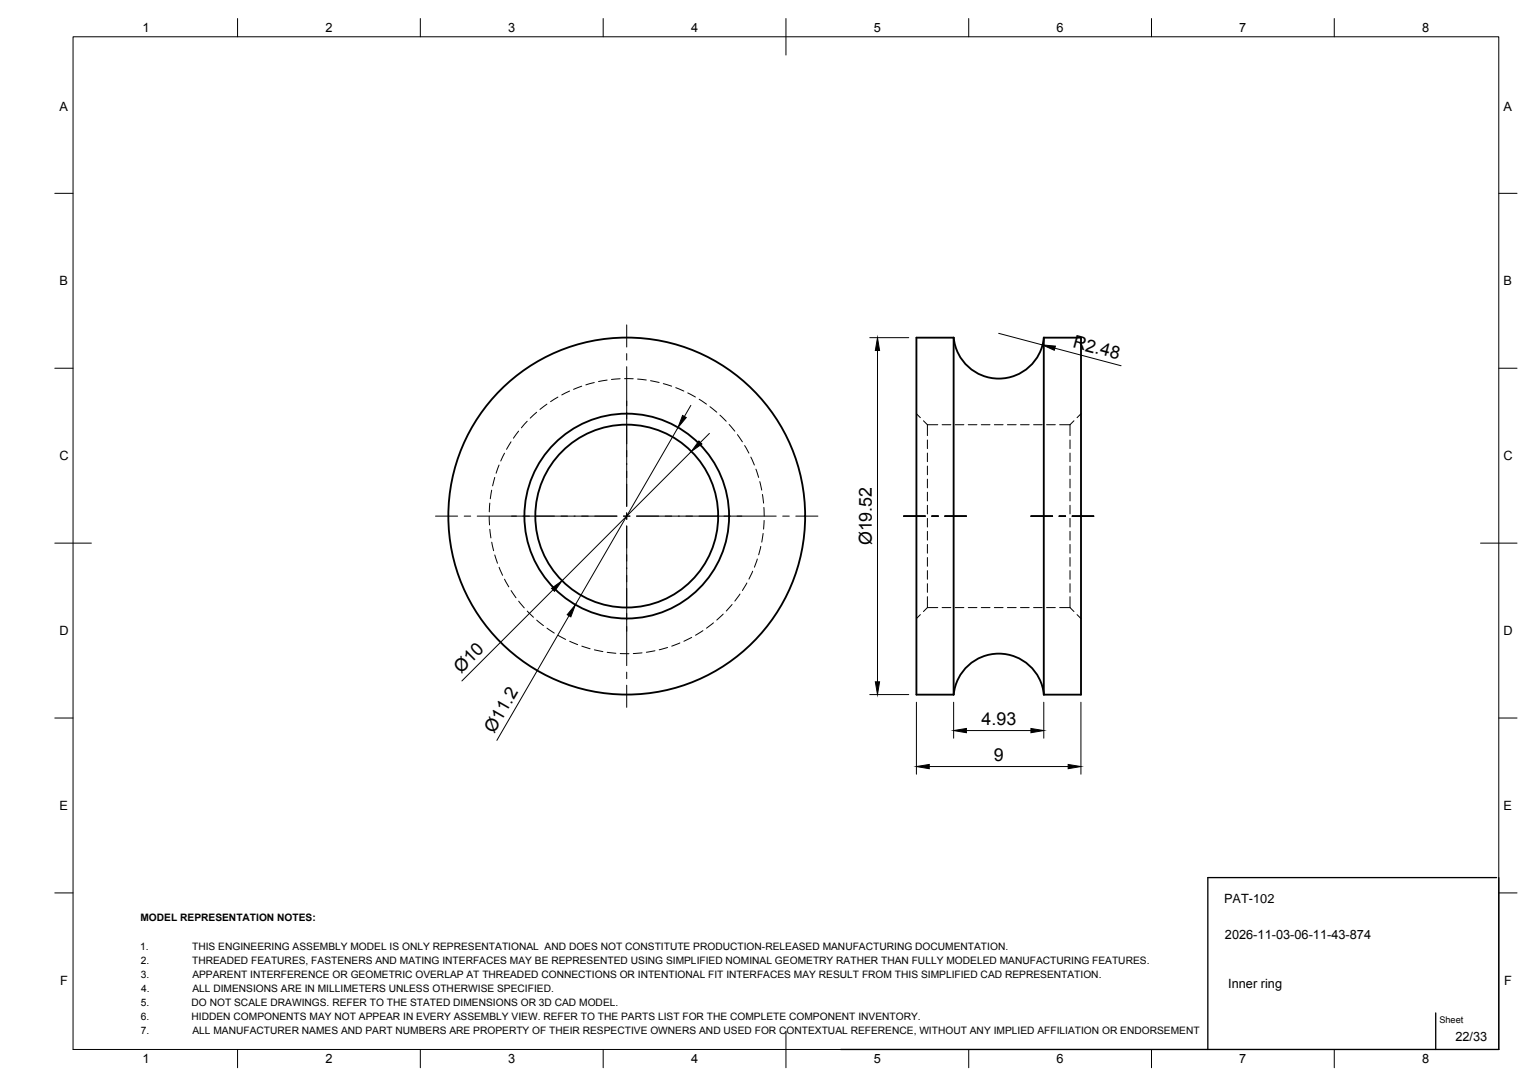
ISO-10303-21;
HEADER;
/* Generated by software containing ST-Developer
 * from STEP Tools, Inc. (www.steptools.com) 
 */

FILE_DESCRIPTION(
/* description */ ('Swing-away clamp arm'),
/* implementation_level */ '2;1');

FILE_NAME(
/* name */ 'Inner ring.step',
/* time_stamp */ '2026-10-28T03:26:03-07:00',
/* author */ (''),
/* organization */ (''),
/* preprocessor_version */ 'ST-DEVELOPER v20.2',
/* originating_system */ 'Autodesk Translation Framework v15.17.0.0',
/* authorisation */ '');

FILE_SCHEMA (('AUTOMOTIVE_DESIGN { 1 0 10303 214 3 1 1 }'));
ENDSEC;

DATA;
#10=MECHANICAL_DESIGN_GEOMETRIC_PRESENTATION_REPRESENTATION('',(#307),#10627);
#27=TOROIDAL_SURFACE('',#5581,1.,0.247676);
#204=CONICAL_SURFACE('',#5592,0.53,0.785398163397448);
#205=CONICAL_SURFACE('',#5599,0.53,0.785398163397448);
#255=SHAPE_REPRESENTATION_RELATIONSHIP('SRR','None',#10755,#281);
#281=ADVANCED_BREP_SHAPE_REPRESENTATION('',(#340),#10614);
#307=STYLED_ITEM('',(#10965),#340);
#340=MANIFOLD_SOLID_BREP('Body1',#4914);
#432=FACE_BOUND('',#1209,.T.);
#433=FACE_BOUND('',#1212,.T.);
#578=PLANE('',#5594);
#579=PLANE('',#5597);
#823=FACE_OUTER_BOUND('',#1204,.T.);
#824=FACE_OUTER_BOUND('',#1205,.T.);
#825=FACE_OUTER_BOUND('',#1206,.T.);
#826=FACE_OUTER_BOUND('',#1207,.T.);
#827=FACE_OUTER_BOUND('',#1208,.T.);
#828=FACE_OUTER_BOUND('',#1210,.T.);
#829=FACE_OUTER_BOUND('',#1211,.T.);
#830=FACE_OUTER_BOUND('',#1213,.T.);
#1204=EDGE_LOOP('',(#4041,#4042,#4043,#4044,#4045,#4046));
#1205=EDGE_LOOP('',(#4047,#4048,#4049,#4050,#4051));
#1206=EDGE_LOOP('',(#4052,#4053,#4054,#4055));
#1207=EDGE_LOOP('',(#4056,#4057,#4058,#4059));
#1208=EDGE_LOOP('',(#4060));
#1209=EDGE_LOOP('',(#4061));
#1210=EDGE_LOOP('',(#4062,#4063,#4064,#4065,#4066));
#1211=EDGE_LOOP('',(#4067));
#1212=EDGE_LOOP('',(#4068));
#1213=EDGE_LOOP('',(#4069,#4070,#4071,#4072));
#1586=LINE('',#9685,#1908);
#1587=LINE('',#9691,#1909);
#1588=LINE('',#9695,#1910);
#1589=LINE('',#9701,#1911);
#1590=LINE('',#9706,#1912);
#1908=VECTOR('',#6835,0.976185);
#1909=VECTOR('',#6842,0.5);
#1910=VECTOR('',#6847,0.53);
#1911=VECTOR('',#6856,0.976185);
#1912=VECTOR('',#6863,0.53);
#2139=CIRCLE('',#5582,0.976185);
#2140=CIRCLE('',#5583,0.976185);
#2141=CIRCLE('',#5584,0.247676);
#2142=CIRCLE('',#5585,0.976185);
#2143=CIRCLE('',#5586,0.976185);
#2144=CIRCLE('',#5588,0.976185);
#2145=CIRCLE('',#5590,0.5);
#2146=CIRCLE('',#5591,0.5);
#2147=CIRCLE('',#5593,0.56);
#2148=CIRCLE('',#5596,0.976185);
#2149=CIRCLE('',#5598,0.56);
#2514=VERTEX_POINT('',#9674);
#2515=VERTEX_POINT('',#9675);
#2516=VERTEX_POINT('',#9678);
#2517=VERTEX_POINT('',#9680);
#2518=VERTEX_POINT('',#9684);
#2519=VERTEX_POINT('',#9688);
#2520=VERTEX_POINT('',#9690);
#2521=VERTEX_POINT('',#9694);
#2522=VERTEX_POINT('',#9699);
#2523=VERTEX_POINT('',#9703);
#3053=EDGE_CURVE('',#2514,#2515,#2139,.T.);
#3054=EDGE_CURVE('',#2515,#2514,#2140,.T.);
#3055=EDGE_CURVE('',#2515,#2516,#2141,.T.);
#3056=EDGE_CURVE('',#2517,#2516,#2142,.T.);
#3057=EDGE_CURVE('',#2516,#2517,#2143,.T.);
#3058=EDGE_CURVE('',#2517,#2518,#1586,.T.);
#3059=EDGE_CURVE('',#2518,#2518,#2144,.T.);
#3060=EDGE_CURVE('',#2519,#2519,#2145,.T.);
#3061=EDGE_CURVE('',#2519,#2520,#1587,.T.);
#3062=EDGE_CURVE('',#2520,#2520,#2146,.T.);
#3063=EDGE_CURVE('',#2520,#2521,#1588,.T.);
#3064=EDGE_CURVE('',#2521,#2521,#2147,.T.);
#3065=EDGE_CURVE('',#2522,#2522,#2148,.T.);
#3066=EDGE_CURVE('',#2522,#2514,#1589,.T.);
#3067=EDGE_CURVE('',#2523,#2523,#2149,.T.);
#3068=EDGE_CURVE('',#2523,#2519,#1590,.T.);
#4041=ORIENTED_EDGE('',*,*,#3053,.F.);
#4042=ORIENTED_EDGE('',*,*,#3054,.F.);
#4043=ORIENTED_EDGE('',*,*,#3055,.T.);
#4044=ORIENTED_EDGE('',*,*,#3056,.F.);
#4045=ORIENTED_EDGE('',*,*,#3057,.F.);
#4046=ORIENTED_EDGE('',*,*,#3055,.F.);
#4047=ORIENTED_EDGE('',*,*,#3056,.T.);
#4048=ORIENTED_EDGE('',*,*,#3057,.T.);
#4049=ORIENTED_EDGE('',*,*,#3058,.T.);
#4050=ORIENTED_EDGE('',*,*,#3059,.T.);
#4051=ORIENTED_EDGE('',*,*,#3058,.F.);
#4052=ORIENTED_EDGE('',*,*,#3060,.T.);
#4053=ORIENTED_EDGE('',*,*,#3061,.T.);
#4054=ORIENTED_EDGE('',*,*,#3062,.F.);
#4055=ORIENTED_EDGE('',*,*,#3061,.F.);
#4056=ORIENTED_EDGE('',*,*,#3062,.T.);
#4057=ORIENTED_EDGE('',*,*,#3063,.T.);
#4058=ORIENTED_EDGE('',*,*,#3064,.F.);
#4059=ORIENTED_EDGE('',*,*,#3063,.F.);
#4060=ORIENTED_EDGE('',*,*,#3059,.F.);
#4061=ORIENTED_EDGE('',*,*,#3064,.T.);
#4062=ORIENTED_EDGE('',*,*,#3065,.F.);
#4063=ORIENTED_EDGE('',*,*,#3066,.T.);
#4064=ORIENTED_EDGE('',*,*,#3053,.T.);
#4065=ORIENTED_EDGE('',*,*,#3054,.T.);
#4066=ORIENTED_EDGE('',*,*,#3066,.F.);
#4067=ORIENTED_EDGE('',*,*,#3065,.T.);
#4068=ORIENTED_EDGE('',*,*,#3067,.F.);
#4069=ORIENTED_EDGE('',*,*,#3067,.T.);
#4070=ORIENTED_EDGE('',*,*,#3068,.T.);
#4071=ORIENTED_EDGE('',*,*,#3060,.F.);
#4072=ORIENTED_EDGE('',*,*,#3068,.F.);
#4559=CYLINDRICAL_SURFACE('',#5587,0.976185);
#4560=CYLINDRICAL_SURFACE('',#5589,0.5);
#4561=CYLINDRICAL_SURFACE('',#5595,0.976185);
#4778=ADVANCED_FACE('',(#823),#27,.F.);
#4779=ADVANCED_FACE('',(#824),#4559,.T.);
#4780=ADVANCED_FACE('',(#825),#4560,.F.);
#4781=ADVANCED_FACE('',(#826),#204,.F.);
#4782=ADVANCED_FACE('',(#827,#432),#578,.T.);
#4783=ADVANCED_FACE('',(#828),#4561,.T.);
#4784=ADVANCED_FACE('',(#829,#433),#579,.T.);
#4785=ADVANCED_FACE('',(#830),#205,.F.);
#4914=CLOSED_SHELL('',(#4778,#4779,#4780,#4781,#4782,#4783,#4784,#4785));
#5580=AXIS2_PLACEMENT_3D('',#9672,#6819,#6820);
#5581=AXIS2_PLACEMENT_3D('',#9673,#6821,#6822);
#5582=AXIS2_PLACEMENT_3D('',#9676,#6823,#6824);
#5583=AXIS2_PLACEMENT_3D('',#9677,#6825,#6826);
#5584=AXIS2_PLACEMENT_3D('',#9679,#6827,#6828);
#5585=AXIS2_PLACEMENT_3D('',#9681,#6829,#6830);
#5586=AXIS2_PLACEMENT_3D('',#9682,#6831,#6832);
#5587=AXIS2_PLACEMENT_3D('',#9683,#6833,#6834);
#5588=AXIS2_PLACEMENT_3D('',#9686,#6836,#6837);
#5589=AXIS2_PLACEMENT_3D('',#9687,#6838,#6839);
#5590=AXIS2_PLACEMENT_3D('',#9689,#6840,#6841);
#5591=AXIS2_PLACEMENT_3D('',#9692,#6843,#6844);
#5592=AXIS2_PLACEMENT_3D('',#9693,#6845,#6846);
#5593=AXIS2_PLACEMENT_3D('',#9696,#6848,#6849);
#5594=AXIS2_PLACEMENT_3D('',#9697,#6850,#6851);
#5595=AXIS2_PLACEMENT_3D('',#9698,#6852,#6853);
#5596=AXIS2_PLACEMENT_3D('',#9700,#6854,#6855);
#5597=AXIS2_PLACEMENT_3D('',#9702,#6857,#6858);
#5598=AXIS2_PLACEMENT_3D('',#9704,#6859,#6860);
#5599=AXIS2_PLACEMENT_3D('',#9705,#6861,#6862);
#6819=DIRECTION('axis',(0.,0.,1.));
#6820=DIRECTION('refdir',(1.,0.,0.));
#6821=DIRECTION('center_axis',(0.,-1.,0.));
#6822=DIRECTION('ref_axis',(0.,0.,-1.));
#6823=DIRECTION('center_axis',(0.,-1.,0.));
#6824=DIRECTION('ref_axis',(1.,0.,0.));
#6825=DIRECTION('center_axis',(0.,-1.,0.));
#6826=DIRECTION('ref_axis',(1.,0.,0.));
#6827=DIRECTION('center_axis',(1.,0.,1.22464679914735E-16));
#6828=DIRECTION('ref_axis',(-1.22464679914735E-16,0.,1.));
#6829=DIRECTION('center_axis',(0.,1.,0.));
#6830=DIRECTION('ref_axis',(1.,0.,0.));
#6831=DIRECTION('center_axis',(0.,1.,0.));
#6832=DIRECTION('ref_axis',(1.,0.,0.));
#6833=DIRECTION('center_axis',(0.,-1.,0.));
#6834=DIRECTION('ref_axis',(1.,0.,0.));
#6835=DIRECTION('',(0.,1.,0.));
#6836=DIRECTION('center_axis',(0.,-1.,0.));
#6837=DIRECTION('ref_axis',(1.,0.,0.));
#6838=DIRECTION('center_axis',(0.,-1.,0.));
#6839=DIRECTION('ref_axis',(1.,0.,0.));
#6840=DIRECTION('center_axis',(0.,-1.,0.));
#6841=DIRECTION('ref_axis',(1.,0.,0.));
#6842=DIRECTION('',(0.,1.,0.));
#6843=DIRECTION('center_axis',(0.,-1.,0.));
#6844=DIRECTION('ref_axis',(1.,0.,0.));
#6845=DIRECTION('center_axis',(0.,1.,0.));
#6846=DIRECTION('ref_axis',(1.,0.,0.));
#6847=DIRECTION('',(-0.707106781186547,0.707106781186548,-8.65956056235493E-17));
#6848=DIRECTION('center_axis',(0.,-1.,0.));
#6849=DIRECTION('ref_axis',(1.,0.,0.));
#6850=DIRECTION('center_axis',(0.,1.,0.));
#6851=DIRECTION('ref_axis',(0.,0.,1.));
#6852=DIRECTION('center_axis',(0.,-1.,0.));
#6853=DIRECTION('ref_axis',(1.,0.,0.));
#6854=DIRECTION('center_axis',(0.,-1.,0.));
#6855=DIRECTION('ref_axis',(1.,0.,0.));
#6856=DIRECTION('',(0.,1.,0.));
#6857=DIRECTION('center_axis',(0.,-1.,0.));
#6858=DIRECTION('ref_axis',(0.,0.,-1.));
#6859=DIRECTION('center_axis',(0.,-1.,0.));
#6860=DIRECTION('ref_axis',(1.,0.,0.));
#6861=DIRECTION('center_axis',(0.,-1.,0.));
#6862=DIRECTION('ref_axis',(1.,0.,0.));
#6863=DIRECTION('',(0.707106781186547,0.707106781186548,8.65956056235493E-17));
#9672=CARTESIAN_POINT('',(0.,0.,0.));
#9673=CARTESIAN_POINT('Origin',(0.,0.,0.));
#9674=CARTESIAN_POINT('',(-0.976185,-0.246528389340863,-1.19548183562566E-16));
#9675=CARTESIAN_POINT('',(-1.19548183562566E-16,-0.246528389340863,0.976185));
#9676=CARTESIAN_POINT('Origin',(0.,-0.246528389340863,0.));
#9677=CARTESIAN_POINT('Origin',(0.,-0.246528389340863,0.));
#9678=CARTESIAN_POINT('',(-1.19548183562566E-16,0.246528389340863,0.976185));
#9679=CARTESIAN_POINT('Origin',(-1.22464679914735E-16,0.,1.));
#9680=CARTESIAN_POINT('',(-0.976185,0.246528389340863,1.19548183562566E-16));
#9681=CARTESIAN_POINT('Origin',(0.,0.246528389340863,0.));
#9682=CARTESIAN_POINT('Origin',(0.,0.246528389340863,0.));
#9683=CARTESIAN_POINT('Origin',(0.,0.,0.));
#9684=CARTESIAN_POINT('',(-0.976185,0.45,-1.19548183562566E-16));
#9685=CARTESIAN_POINT('',(-0.976185,0.,-1.19548183562566E-16));
#9686=CARTESIAN_POINT('Origin',(0.,0.45,0.));
#9687=CARTESIAN_POINT('Origin',(0.,0.,0.));
#9688=CARTESIAN_POINT('',(-0.5,-0.39,-6.12323399573677E-17));
#9689=CARTESIAN_POINT('Origin',(0.,-0.39,0.));
#9690=CARTESIAN_POINT('',(-0.5,0.39,-6.12323399573677E-17));
#9691=CARTESIAN_POINT('',(-0.5,0.,-6.12323399573677E-17));
#9692=CARTESIAN_POINT('Origin',(0.,0.39,0.));
#9693=CARTESIAN_POINT('Origin',(0.,0.42,0.));
#9694=CARTESIAN_POINT('',(-0.56,0.45,-6.85802207522518E-17));
#9695=CARTESIAN_POINT('',(-0.53,0.42,-6.49062803548097E-17));
#9696=CARTESIAN_POINT('Origin',(0.,0.45,0.));
#9697=CARTESIAN_POINT('Origin',(0.976185,0.45,0.));
#9698=CARTESIAN_POINT('Origin',(0.,0.,0.));
#9699=CARTESIAN_POINT('',(-0.976185,-0.45,-1.19548183562566E-16));
#9700=CARTESIAN_POINT('Origin',(0.,-0.45,0.));
#9701=CARTESIAN_POINT('',(-0.976185,0.,-1.19548183562566E-16));
#9702=CARTESIAN_POINT('Origin',(0.56,-0.45,0.));
#9703=CARTESIAN_POINT('',(-0.56,-0.45,-6.85802207522518E-17));
#9704=CARTESIAN_POINT('Origin',(0.,-0.45,0.));
#9705=CARTESIAN_POINT('Origin',(0.,-0.42,0.));
#9706=CARTESIAN_POINT('',(-0.53,-0.42,-6.49062803548097E-17));
#10582=UNCERTAINTY_MEASURE_WITH_UNIT(LENGTH_MEASURE(0.001),#10628,
'DISTANCE_ACCURACY_VALUE',
'Maximum model space distance between geometric entities at asserted c
onnectivities');
#10595=UNCERTAINTY_MEASURE_WITH_UNIT(LENGTH_MEASURE(0.001),#10628,
'DISTANCE_ACCURACY_VALUE',
'Maximum model space distance between geometric entities at asserted c
onnectivities');
#10614=(
GEOMETRIC_REPRESENTATION_CONTEXT(3)
GLOBAL_UNCERTAINTY_ASSIGNED_CONTEXT((#10582))
GLOBAL_UNIT_ASSIGNED_CONTEXT((#10628,#10630,#10631))
REPRESENTATION_CONTEXT('','3D')
);
#10627=(
GEOMETRIC_REPRESENTATION_CONTEXT(3)
GLOBAL_UNCERTAINTY_ASSIGNED_CONTEXT((#10595))
GLOBAL_UNIT_ASSIGNED_CONTEXT((#10628,#10630,#10631))
REPRESENTATION_CONTEXT('','3D')
);
#10628=(
LENGTH_UNIT()
NAMED_UNIT(*)
SI_UNIT(.CENTI.,.METRE.)
);
#10630=(
NAMED_UNIT(*)
PLANE_ANGLE_UNIT()
SI_UNIT($,.RADIAN.)
);
#10631=(
NAMED_UNIT(*)
SI_UNIT($,.STERADIAN.)
SOLID_ANGLE_UNIT()
);
#10650=SHAPE_DEFINITION_REPRESENTATION(#10691,#10755);
#10691=PRODUCT_DEFINITION_SHAPE('',$,#10787);
#10755=SHAPE_REPRESENTATION('',(#5580),#10614);
#10768=PRODUCT_DEFINITION_CONTEXT('part definition',#10863,'design');
#10787=PRODUCT_DEFINITION('Inner ring','Inner ring',#10818,#10768);
#10818=PRODUCT_DEFINITION_FORMATION('',$,#10883);
#10863=APPLICATION_CONTEXT(
'Core Data for Automotive Mechanical Design Process');
#10864=PRODUCT_CONTEXT('part definition',#10863,'mechanical');
#10883=PRODUCT('Inner ring','Inner ring','Inner ring',(#10864));
#10959=COLOUR_RGB('Grey',0.48,0.52,0.57);
#10960=FILL_AREA_STYLE_COLOUR('',#10959);
#10961=FILL_AREA_STYLE('',(#10960));
#10962=SURFACE_STYLE_FILL_AREA(#10961);
#10963=SURFACE_SIDE_STYLE('',(#10962));
#10964=SURFACE_STYLE_USAGE(.BOTH.,#10963);
#10965=PRESENTATION_STYLE_ASSIGNMENT((#10964));
ENDSEC;
END-ISO-10303-21;
